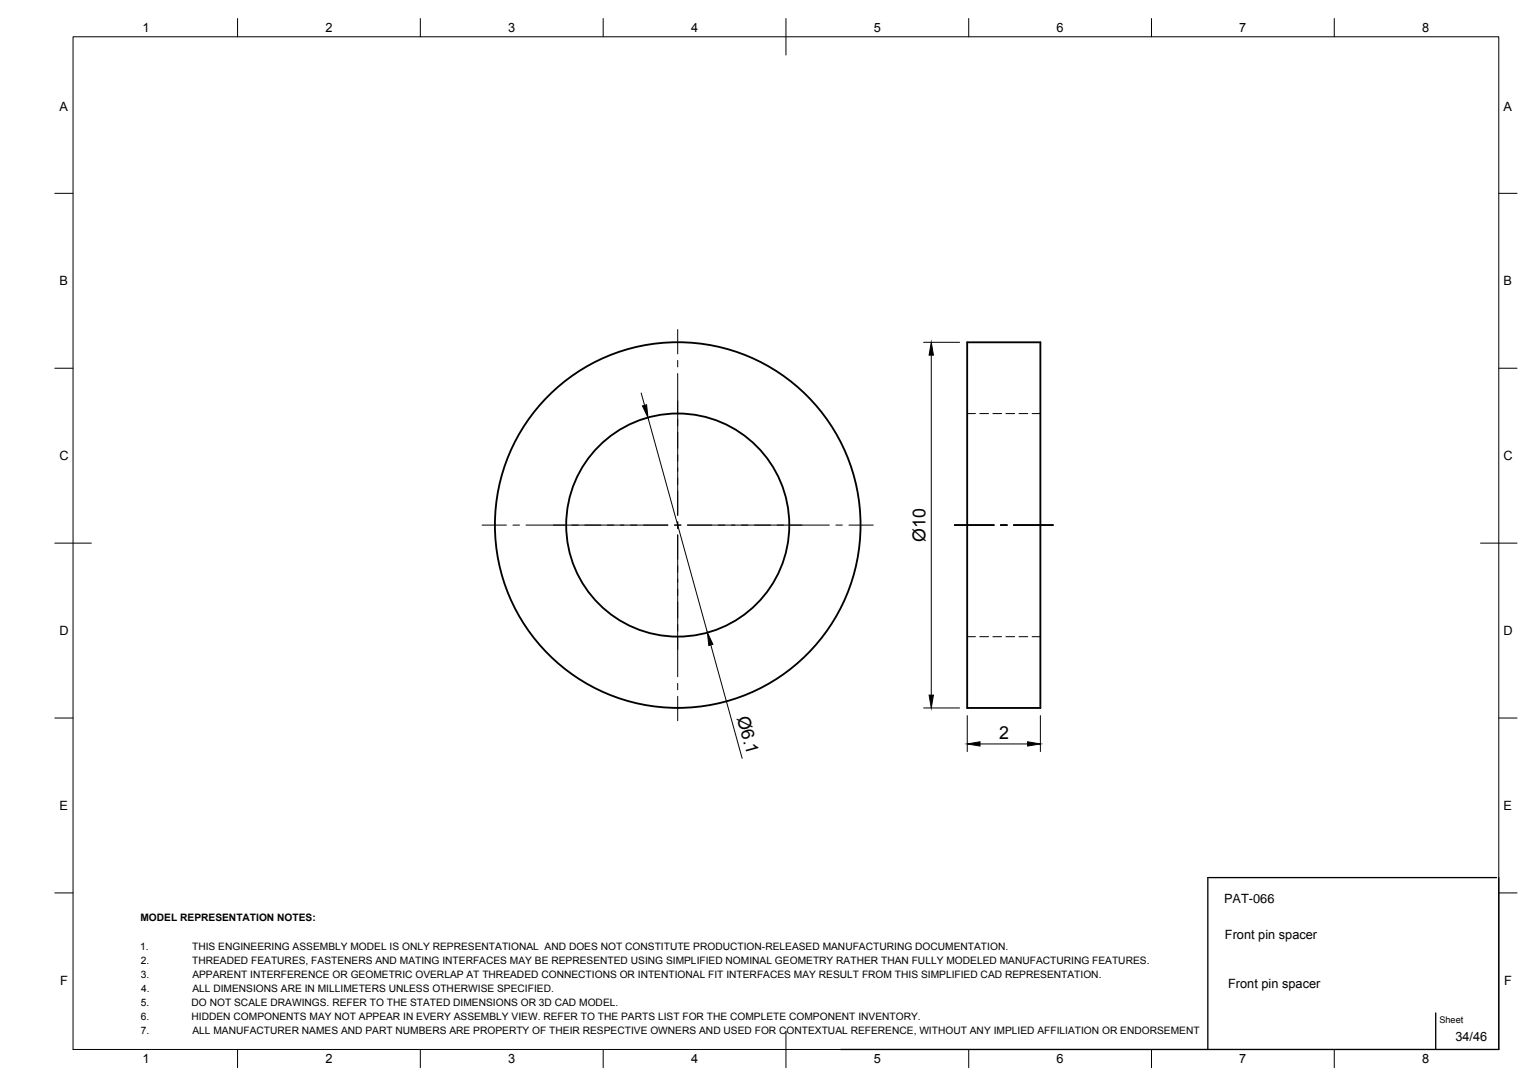
ISO-10303-21;
HEADER;
/* Generated by software containing ST-Developer
 * from STEP Tools, Inc. (www.steptools.com) 
 */

FILE_DESCRIPTION(
/* description */ ('Lever-operated bar clamp (toggle)'),
/* implementation_level */ '2;1');

FILE_NAME(
/* name */ 'Front pin spacer.step',
/* time_stamp */ '2026-10-28T03:25:02-07:00',
/* author */ (''),
/* organization */ (''),
/* preprocessor_version */ 'ST-DEVELOPER v20.2',
/* originating_system */ 'Autodesk Translation Framework v15.17.0.0',
/* authorisation */ '');

FILE_SCHEMA (('AUTOMOTIVE_DESIGN { 1 0 10303 214 3 1 1 }'));
ENDSEC;

DATA;
#10=MECHANICAL_DESIGN_GEOMETRIC_PRESENTATION_REPRESENTATION('',(#443),#12413);
#359=SHAPE_REPRESENTATION_RELATIONSHIP('SRR','None',#12601,#397);
#397=ADVANCED_BREP_SHAPE_REPRESENTATION('',(#488),#12398);
#443=STYLED_ITEM('',(#12869),#488);
#488=MANIFOLD_SOLID_BREP('Body1',#6604);
#627=FACE_BOUND('',#1714,.T.);
#628=FACE_BOUND('',#1716,.T.);
#810=PLANE('',#7643);
#811=PLANE('',#7644);
#1178=FACE_OUTER_BOUND('',#1711,.T.);
#1179=FACE_OUTER_BOUND('',#1712,.T.);
#1180=FACE_OUTER_BOUND('',#1713,.T.);
#1181=FACE_OUTER_BOUND('',#1715,.T.);
#1711=EDGE_LOOP('',(#5587,#5588,#5589,#5590));
#1712=EDGE_LOOP('',(#5591,#5592,#5593,#5594));
#1713=EDGE_LOOP('',(#5595));
#1714=EDGE_LOOP('',(#5596));
#1715=EDGE_LOOP('',(#5597));
#1716=EDGE_LOOP('',(#5598));
#2142=LINE('',#11754,#2583);
#2143=LINE('',#11760,#2584);
#2583=VECTOR('',#9385,0.305);
#2584=VECTOR('',#9392,0.5);
#3003=CIRCLE('',#7638,0.305);
#3004=CIRCLE('',#7639,0.305);
#3005=CIRCLE('',#7641,0.5);
#3006=CIRCLE('',#7642,0.5);
#3470=VERTEX_POINT('',#11751);
#3471=VERTEX_POINT('',#11753);
#3472=VERTEX_POINT('',#11757);
#3473=VERTEX_POINT('',#11759);
#4198=EDGE_CURVE('',#3470,#3470,#3003,.T.);
#4199=EDGE_CURVE('',#3470,#3471,#2142,.T.);
#4200=EDGE_CURVE('',#3471,#3471,#3004,.T.);
#4201=EDGE_CURVE('',#3472,#3472,#3005,.T.);
#4202=EDGE_CURVE('',#3472,#3473,#2143,.T.);
#4203=EDGE_CURVE('',#3473,#3473,#3006,.T.);
#5587=ORIENTED_EDGE('',*,*,#4198,.F.);
#5588=ORIENTED_EDGE('',*,*,#4199,.T.);
#5589=ORIENTED_EDGE('',*,*,#4200,.T.);
#5590=ORIENTED_EDGE('',*,*,#4199,.F.);
#5591=ORIENTED_EDGE('',*,*,#4201,.F.);
#5592=ORIENTED_EDGE('',*,*,#4202,.T.);
#5593=ORIENTED_EDGE('',*,*,#4203,.T.);
#5594=ORIENTED_EDGE('',*,*,#4202,.F.);
#5595=ORIENTED_EDGE('',*,*,#4201,.T.);
#5596=ORIENTED_EDGE('',*,*,#4198,.T.);
#5597=ORIENTED_EDGE('',*,*,#4203,.F.);
#5598=ORIENTED_EDGE('',*,*,#4200,.F.);
#6135=CYLINDRICAL_SURFACE('',#7637,0.305);
#6136=CYLINDRICAL_SURFACE('',#7640,0.5);
#6453=ADVANCED_FACE('',(#1178),#6135,.F.);
#6454=ADVANCED_FACE('',(#1179),#6136,.T.);
#6455=ADVANCED_FACE('',(#1180,#627),#810,.T.);
#6456=ADVANCED_FACE('',(#1181,#628),#811,.F.);
#6604=CLOSED_SHELL('',(#6453,#6454,#6455,#6456));
#7636=AXIS2_PLACEMENT_3D('',#11749,#9379,#9380);
#7637=AXIS2_PLACEMENT_3D('',#11750,#9381,#9382);
#7638=AXIS2_PLACEMENT_3D('',#11752,#9383,#9384);
#7639=AXIS2_PLACEMENT_3D('',#11755,#9386,#9387);
#7640=AXIS2_PLACEMENT_3D('',#11756,#9388,#9389);
#7641=AXIS2_PLACEMENT_3D('',#11758,#9390,#9391);
#7642=AXIS2_PLACEMENT_3D('',#11761,#9393,#9394);
#7643=AXIS2_PLACEMENT_3D('',#11762,#9395,#9396);
#7644=AXIS2_PLACEMENT_3D('',#11763,#9397,#9398);
#9379=DIRECTION('axis',(0.,0.,1.));
#9380=DIRECTION('refdir',(1.,0.,0.));
#9381=DIRECTION('center_axis',(0.,1.,0.));
#9382=DIRECTION('ref_axis',(1.,0.,0.));
#9383=DIRECTION('center_axis',(0.,-1.,0.));
#9384=DIRECTION('ref_axis',(1.,0.,0.));
#9385=DIRECTION('',(0.,-1.,0.));
#9386=DIRECTION('center_axis',(0.,-1.,0.));
#9387=DIRECTION('ref_axis',(1.,0.,0.));
#9388=DIRECTION('center_axis',(0.,1.,0.));
#9389=DIRECTION('ref_axis',(1.,0.,0.));
#9390=DIRECTION('center_axis',(0.,1.,0.));
#9391=DIRECTION('ref_axis',(1.,0.,0.));
#9392=DIRECTION('',(0.,-1.,0.));
#9393=DIRECTION('center_axis',(0.,1.,0.));
#9394=DIRECTION('ref_axis',(1.,0.,0.));
#9395=DIRECTION('center_axis',(0.,1.,0.));
#9396=DIRECTION('ref_axis',(1.,0.,0.));
#9397=DIRECTION('center_axis',(0.,1.,0.));
#9398=DIRECTION('ref_axis',(1.,0.,0.));
#11749=CARTESIAN_POINT('',(0.,0.,0.));
#11750=CARTESIAN_POINT('Origin',(-2.82632109303527,-5.7,8.79263101785268));
#11751=CARTESIAN_POINT('',(-3.13132109303527,-5.5,8.79263101785268));
#11752=CARTESIAN_POINT('Origin',(-2.82632109303527,-5.5,8.79263101785268));
#11753=CARTESIAN_POINT('',(-3.13132109303527,-5.7,8.79263101785268));
#11754=CARTESIAN_POINT('',(-3.13132109303527,-5.7,8.79263101785268));
#11755=CARTESIAN_POINT('Origin',(-2.82632109303527,-5.7,8.79263101785268));
#11756=CARTESIAN_POINT('Origin',(-2.82632109303527,-5.7,8.79263101785268));
#11757=CARTESIAN_POINT('',(-3.32632109303527,-5.5,8.79263101785268));
#11758=CARTESIAN_POINT('Origin',(-2.82632109303527,-5.5,8.79263101785268));
#11759=CARTESIAN_POINT('',(-3.32632109303527,-5.7,8.79263101785268));
#11760=CARTESIAN_POINT('',(-3.32632109303527,-5.7,8.79263101785268));
#11761=CARTESIAN_POINT('Origin',(-2.82632109303527,-5.7,8.79263101785268));
#11762=CARTESIAN_POINT('Origin',(-2.82632109303527,-5.5,8.79263101785268));
#11763=CARTESIAN_POINT('Origin',(-2.82632109303527,-5.7,8.79263101785268));
#12352=UNCERTAINTY_MEASURE_WITH_UNIT(LENGTH_MEASURE(0.001),#12414,
'DISTANCE_ACCURACY_VALUE',
'Maximum model space distance between geometric entities at asserted c
onnectivities');
#12367=UNCERTAINTY_MEASURE_WITH_UNIT(LENGTH_MEASURE(0.001),#12414,
'DISTANCE_ACCURACY_VALUE',
'Maximum model space distance between geometric entities at asserted c
onnectivities');
#12398=(
GEOMETRIC_REPRESENTATION_CONTEXT(3)
GLOBAL_UNCERTAINTY_ASSIGNED_CONTEXT((#12352))
GLOBAL_UNIT_ASSIGNED_CONTEXT((#12414,#12416,#12417))
REPRESENTATION_CONTEXT('','3D')
);
#12413=(
GEOMETRIC_REPRESENTATION_CONTEXT(3)
GLOBAL_UNCERTAINTY_ASSIGNED_CONTEXT((#12367))
GLOBAL_UNIT_ASSIGNED_CONTEXT((#12414,#12416,#12417))
REPRESENTATION_CONTEXT('','3D')
);
#12414=(
LENGTH_UNIT()
NAMED_UNIT(*)
SI_UNIT(.CENTI.,.METRE.)
);
#12416=(
NAMED_UNIT(*)
PLANE_ANGLE_UNIT()
SI_UNIT($,.RADIAN.)
);
#12417=(
NAMED_UNIT(*)
SI_UNIT($,.STERADIAN.)
SOLID_ANGLE_UNIT()
);
#12448=SHAPE_DEFINITION_REPRESENTATION(#12500,#12601);
#12500=PRODUCT_DEFINITION_SHAPE('',$,#12647);
#12601=SHAPE_REPRESENTATION('',(#7636),#12398);
#12616=PRODUCT_DEFINITION_CONTEXT('part definition',#12753,'design');
#12647=PRODUCT_DEFINITION('Front pin spacer','Front pin spacer',#12692,
#12616);
#12692=PRODUCT_DEFINITION_FORMATION('',$,#12785);
#12753=APPLICATION_CONTEXT(
'Core Data for Automotive Mechanical Design Process');
#12754=PRODUCT_CONTEXT('part definition',#12753,'mechanical');
#12785=PRODUCT('Front pin spacer','Front pin spacer','Front pin spacer',
(#12754));
#12863=COLOUR_RGB('Grey',0.48,0.52,0.57);
#12864=FILL_AREA_STYLE_COLOUR('',#12863);
#12865=FILL_AREA_STYLE('',(#12864));
#12866=SURFACE_STYLE_FILL_AREA(#12865);
#12867=SURFACE_SIDE_STYLE('',(#12866));
#12868=SURFACE_STYLE_USAGE(.BOTH.,#12867);
#12869=PRESENTATION_STYLE_ASSIGNMENT((#12868));
ENDSEC;
END-ISO-10303-21;
